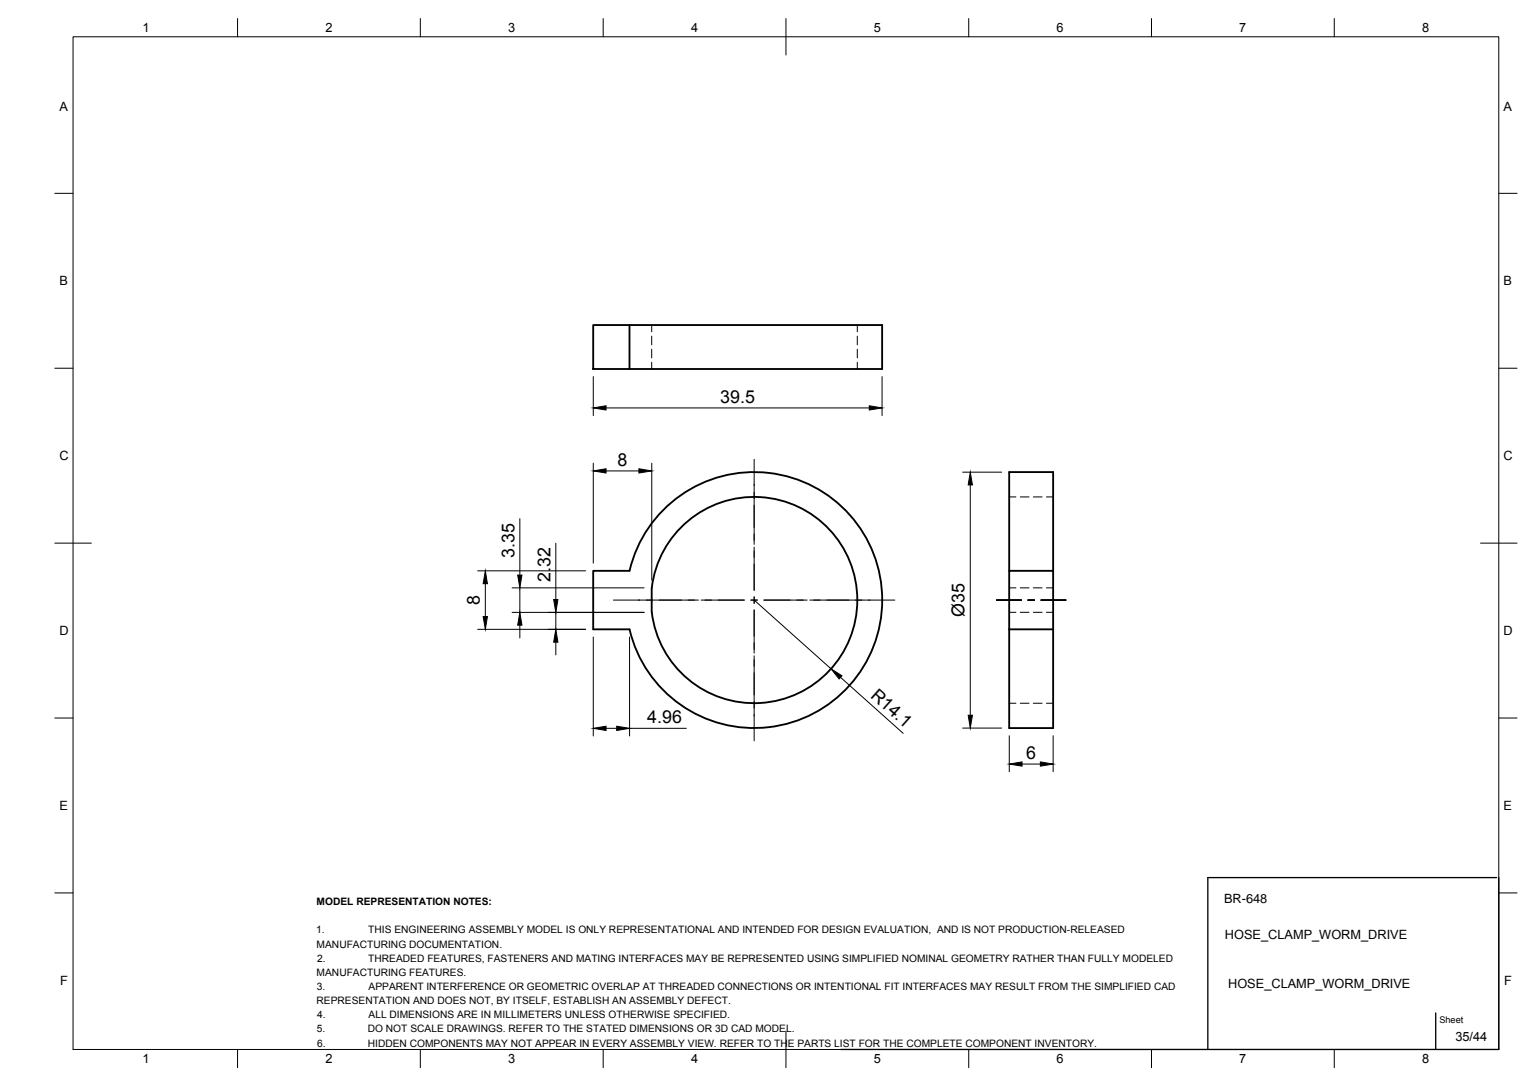
ISO-10303-21;
HEADER;
FILE_DESCRIPTION((''),'2;1');
FILE_NAME('HOSE_CLAMP_WORM_DRIVE.step','2026-10-01T22:05:39-07:00',(''),(''),'','','');
FILE_SCHEMA (('AUTOMOTIVE_DESIGN { 1 0 10303 214 3 1 1 }'));
ENDSEC;
DATA;
#10=MECHANICAL_DESIGN_GEOMETRIC_PRESENTATION_REPRESENTATION('',(#633),#24628);
#549=SHAPE_REPRESENTATION_RELATIONSHIP('SRR','None',#24822,#591) ;
#591=ADVANCED_BREP_SHAPE_REPRESENTATION('',(#672),#24612) ;
#633=STYLED_ITEM('',(#25034),#672) ;
#672=MANIFOLD_SOLID_BREP('HOSE_CLAMP_WORM_DRIVE',#13175) ;
#904=FACE_BOUND('',#4596,.T.) ;
#905=FACE_BOUND('',#4600,.T.) ;
#1679=LINE('',#23705,#2515) ;
#1680=LINE('',#23707,#2516) ;
#1681=LINE('',#23709,#2517) ;
#1682=LINE('',#23710,#2518) ;
#1683=LINE('',#23714,#2519) ;
#1684=LINE('',#23716,#2520) ;
#1685=LINE('',#23718,#2521) ;
#1686=LINE('',#23719,#2522) ;
#1687=LINE('',#23723,#2523) ;
#1688=LINE('',#23725,#2524) ;
#1689=LINE('',#23727,#2525) ;
#1690=LINE('',#23728,#2526) ;
#1691=LINE('',#23730,#2527) ;
#1692=LINE('',#23731,#2528) ;
#2515=VECTOR('',#19054,1.) ;
#2516=VECTOR('',#19055,1.) ;
#2517=VECTOR('',#19056,1.) ;
#2518=VECTOR('',#19057,1.) ;
#2519=VECTOR('',#19060,1.) ;
#2520=VECTOR('',#19061,1.) ;
#2521=VECTOR('',#19062,1.) ;
#2522=VECTOR('',#19063,1.) ;
#2523=VECTOR('',#19066,1.) ;
#2524=VECTOR('',#19067,1.) ;
#2525=VECTOR('',#19068,1.) ;
#2526=VECTOR('',#19069,1.) ;
#2527=VECTOR('',#19072,1.) ;
#2528=VECTOR('',#19073,1.) ;
#2913=CYLINDRICAL_SURFACE('',#15151,1.41) ;
#2914=CYLINDRICAL_SURFACE('',#15153,1.75) ;
#3606=FACE_OUTER_BOUND('',#4591,.T.) ;
#3607=FACE_OUTER_BOUND('',#4592,.T.) ;
#3608=FACE_OUTER_BOUND('',#4593,.T.) ;
#3609=FACE_OUTER_BOUND('',#4594,.T.) ;
#3610=FACE_OUTER_BOUND('',#4595,.T.) ;
#3611=FACE_OUTER_BOUND('',#4597,.T.) ;
#3612=FACE_OUTER_BOUND('',#4598,.T.) ;
#3613=FACE_OUTER_BOUND('',#4599,.T.) ;
#4591=EDGE_LOOP('',(#11495,#11496,#11497,#11498)) ;
#4592=EDGE_LOOP('',(#11499,#11500,#11501,#11502)) ;
#4593=EDGE_LOOP('',(#11503,#11504,#11505,#11506)) ;
#4594=EDGE_LOOP('',(#11507,#11508,#11509,#11510)) ;
#4595=EDGE_LOOP('',(#11511,#11512,#11513,#11514)) ;
#4596=EDGE_LOOP('',(#11515,#11516)) ;
#4597=EDGE_LOOP('',(#11517,#11518,#11519,#11520)) ;
#4598=EDGE_LOOP('',(#11521,#11522,#11523,#11524)) ;
#4599=EDGE_LOOP('',(#11525,#11526,#11527,#11528)) ;
#4600=EDGE_LOOP('',(#11529,#11530)) ;
#5461=CIRCLE('',#15149,1.75) ;
#5462=CIRCLE('',#15150,1.41) ;
#5463=CIRCLE('',#15152,1.41) ;
#5464=CIRCLE('',#15154,1.75) ;
#6567=VERTEX_POINT('',#23703) ;
#6568=VERTEX_POINT('',#23704) ;
#6569=VERTEX_POINT('',#23706) ;
#6570=VERTEX_POINT('',#23708) ;
#6571=VERTEX_POINT('',#23712) ;
#6572=VERTEX_POINT('',#23713) ;
#6573=VERTEX_POINT('',#23715) ;
#6574=VERTEX_POINT('',#23717) ;
#6575=VERTEX_POINT('',#23721) ;
#6576=VERTEX_POINT('',#23722) ;
#6577=VERTEX_POINT('',#23724) ;
#6578=VERTEX_POINT('',#23726) ;
#8237=EDGE_CURVE('',#6567,#6568,#1679,.T.) ;
#8238=EDGE_CURVE('',#6569,#6567,#1680,.T.) ;
#8239=EDGE_CURVE('',#6570,#6569,#1681,.T.) ;
#8240=EDGE_CURVE('',#6568,#6570,#1682,.T.) ;
#8241=EDGE_CURVE('',#6571,#6572,#1683,.T.) ;
#8242=EDGE_CURVE('',#6573,#6571,#1684,.T.) ;
#8243=EDGE_CURVE('',#6574,#6573,#1685,.T.) ;
#8244=EDGE_CURVE('',#6572,#6574,#1686,.T.) ;
#8245=EDGE_CURVE('',#6575,#6576,#1687,.T.) ;
#8246=EDGE_CURVE('',#6577,#6575,#1688,.T.) ;
#8247=EDGE_CURVE('',#6577,#6578,#1689,.T.) ;
#8248=EDGE_CURVE('',#6576,#6578,#1690,.T.) ;
#8249=EDGE_CURVE('',#6578,#6569,#1691,.T.) ;
#8250=EDGE_CURVE('',#6570,#6577,#1692,.T.) ;
#8251=EDGE_CURVE('',#6567,#6576,#5461,.T.) ;
#8252=EDGE_CURVE('',#6574,#6572,#5462,.T.) ;
#8253=EDGE_CURVE('',#6571,#6573,#5463,.T.) ;
#8254=EDGE_CURVE('',#6575,#6568,#5464,.T.) ;
#11495=ORIENTED_EDGE('',*,*,#8237,.F.) ;
#11496=ORIENTED_EDGE('',*,*,#8238,.F.) ;
#11497=ORIENTED_EDGE('',*,*,#8239,.F.) ;
#11498=ORIENTED_EDGE('',*,*,#8240,.F.) ;
#11499=ORIENTED_EDGE('',*,*,#8241,.F.) ;
#11500=ORIENTED_EDGE('',*,*,#8242,.F.) ;
#11501=ORIENTED_EDGE('',*,*,#8243,.F.) ;
#11502=ORIENTED_EDGE('',*,*,#8244,.F.) ;
#11503=ORIENTED_EDGE('',*,*,#8245,.F.) ;
#11504=ORIENTED_EDGE('',*,*,#8246,.F.) ;
#11505=ORIENTED_EDGE('',*,*,#8247,.T.) ;
#11506=ORIENTED_EDGE('',*,*,#8248,.F.) ;
#11507=ORIENTED_EDGE('',*,*,#8239,.T.) ;
#11508=ORIENTED_EDGE('',*,*,#8249,.F.) ;
#11509=ORIENTED_EDGE('',*,*,#8247,.F.) ;
#11510=ORIENTED_EDGE('',*,*,#8250,.F.) ;
#11511=ORIENTED_EDGE('',*,*,#8251,.T.) ;
#11512=ORIENTED_EDGE('',*,*,#8248,.T.) ;
#11513=ORIENTED_EDGE('',*,*,#8249,.T.) ;
#11514=ORIENTED_EDGE('',*,*,#8238,.T.) ;
#11515=ORIENTED_EDGE('',*,*,#8252,.T.) ;
#11516=ORIENTED_EDGE('',*,*,#8244,.T.) ;
#11517=ORIENTED_EDGE('',*,*,#8241,.T.) ;
#11518=ORIENTED_EDGE('',*,*,#8252,.F.) ;
#11519=ORIENTED_EDGE('',*,*,#8243,.T.) ;
#11520=ORIENTED_EDGE('',*,*,#8253,.F.) ;
#11521=ORIENTED_EDGE('',*,*,#8237,.T.) ;
#11522=ORIENTED_EDGE('',*,*,#8254,.F.) ;
#11523=ORIENTED_EDGE('',*,*,#8245,.T.) ;
#11524=ORIENTED_EDGE('',*,*,#8251,.F.) ;
#11525=ORIENTED_EDGE('',*,*,#8240,.T.) ;
#11526=ORIENTED_EDGE('',*,*,#8250,.T.) ;
#11527=ORIENTED_EDGE('',*,*,#8246,.T.) ;
#11528=ORIENTED_EDGE('',*,*,#8254,.T.) ;
#11529=ORIENTED_EDGE('',*,*,#8253,.T.) ;
#11530=ORIENTED_EDGE('',*,*,#8242,.T.) ;
#12275=PLANE('',#15144) ;
#12276=PLANE('',#15145) ;
#12277=PLANE('',#15146) ;
#12278=PLANE('',#15147) ;
#12279=PLANE('',#15148) ;
#12280=PLANE('',#15155) ;
#13001=ADVANCED_FACE('',(#3606),#12275,.F.) ;
#13002=ADVANCED_FACE('',(#3607),#12276,.F.) ;
#13003=ADVANCED_FACE('',(#3608),#12277,.F.) ;
#13004=ADVANCED_FACE('',(#3609),#12278,.F.) ;
#13005=ADVANCED_FACE('',(#3610,#904),#12279,.T.) ;
#13006=ADVANCED_FACE('',(#3611),#2913,.F.) ;
#13007=ADVANCED_FACE('',(#3612),#2914,.T.) ;
#13008=ADVANCED_FACE('',(#3613,#905),#12280,.T.) ;
#13175=CLOSED_SHELL('',(#13001,#13002,#13003,#13004,#13005,#13006,#13007,
#13008)) ;
#15143=AXIS2_PLACEMENT_3D('',#23701,#19050,#19051) ;
#15144=AXIS2_PLACEMENT_3D('',#23702,#19052,#19053) ;
#15145=AXIS2_PLACEMENT_3D('',#23711,#19058,#19059) ;
#15146=AXIS2_PLACEMENT_3D('',#23720,#19064,#19065) ;
#15147=AXIS2_PLACEMENT_3D('',#23729,#19070,#19071) ;
#15148=AXIS2_PLACEMENT_3D('',#23732,#19074,#19075) ;
#15149=AXIS2_PLACEMENT_3D('',#23733,#19076,#19077) ;
#15150=AXIS2_PLACEMENT_3D('',#23734,#19078,#19079) ;
#15151=AXIS2_PLACEMENT_3D('',#23735,#19080,#19081) ;
#15152=AXIS2_PLACEMENT_3D('',#23736,#19082,#19083) ;
#15153=AXIS2_PLACEMENT_3D('',#23737,#19084,#19085) ;
#15154=AXIS2_PLACEMENT_3D('',#23738,#19086,#19087) ;
#15155=AXIS2_PLACEMENT_3D('',#23739,#19088,#19089) ;
#19050=DIRECTION('axis',(0.,0.,1.)) ;
#19051=DIRECTION('refdir',(1.,0.,0.)) ;
#19052=DIRECTION('center_axis',(0.,1.,0.)) ;
#19053=DIRECTION('ref_axis',(0.,0.,1.)) ;
#19054=DIRECTION('',(0.,0.,1.)) ;
#19055=DIRECTION('',(-1.,0.,0.)) ;
#19056=DIRECTION('',(0.,0.,-1.)) ;
#19057=DIRECTION('',(1.,0.,0.)) ;
#19058=DIRECTION('center_axis',(1.,0.,0.)) ;
#19059=DIRECTION('ref_axis',(0.,0.,-1.)) ;
#19060=DIRECTION('',(0.,0.,-1.)) ;
#19061=DIRECTION('',(0.,-1.,0.)) ;
#19062=DIRECTION('',(0.,0.,1.)) ;
#19063=DIRECTION('',(0.,1.,0.)) ;
#19064=DIRECTION('center_axis',(0.,-1.,0.)) ;
#19065=DIRECTION('ref_axis',(0.,0.,-1.)) ;
#19066=DIRECTION('',(0.,0.,-1.)) ;
#19067=DIRECTION('',(-1.,0.,0.)) ;
#19068=DIRECTION('',(0.,0.,-1.)) ;
#19069=DIRECTION('',(1.,0.,0.)) ;
#19070=DIRECTION('center_axis',(-1.,0.,0.)) ;
#19071=DIRECTION('ref_axis',(0.,0.,1.)) ;
#19072=DIRECTION('',(0.,-1.,0.)) ;
#19073=DIRECTION('',(0.,1.,0.)) ;
#19074=DIRECTION('center_axis',(0.,0.,-1.)) ;
#19075=DIRECTION('ref_axis',(-1.,0.,0.)) ;
#19076=DIRECTION('center_axis',(0.,0.,-1.)) ;
#19077=DIRECTION('ref_axis',(1.,0.,0.)) ;
#19078=DIRECTION('center_axis',(0.,0.,1.)) ;
#19079=DIRECTION('ref_axis',(1.,0.,0.)) ;
#19080=DIRECTION('center_axis',(0.,0.,1.)) ;
#19081=DIRECTION('ref_axis',(-1.,-1.22464679914735E-16,0.)) ;
#19082=DIRECTION('center_axis',(0.,0.,-1.)) ;
#19083=DIRECTION('ref_axis',(1.,0.,0.)) ;
#19084=DIRECTION('center_axis',(0.,0.,1.)) ;
#19085=DIRECTION('ref_axis',(-1.,-1.22464679914735E-16,0.)) ;
#19086=DIRECTION('center_axis',(0.,0.,1.)) ;
#19087=DIRECTION('ref_axis',(1.,0.,0.)) ;
#19088=DIRECTION('center_axis',(0.,0.,1.)) ;
#19089=DIRECTION('ref_axis',(1.,0.,0.)) ;
#23701=CARTESIAN_POINT('',(0.,0.,0.)) ;
#23702=CARTESIAN_POINT('Origin',(-21.2,-2.2,-6.9)) ;
#23703=CARTESIAN_POINT('',(-21.2963274962599,-2.2,-7.2)) ;
#23704=CARTESIAN_POINT('',(-21.2963274962599,-2.2,-6.6)) ;
#23705=CARTESIAN_POINT('',(-21.2963274962599,-2.2,-6.9)) ;
#23706=CARTESIAN_POINT('',(-20.8,-2.2,-7.2)) ;
#23707=CARTESIAN_POINT('',(-21.2,-2.2,-7.2)) ;
#23708=CARTESIAN_POINT('',(-20.8,-2.2,-6.6)) ;
#23709=CARTESIAN_POINT('',(-20.8,-2.2,-6.9)) ;
#23710=CARTESIAN_POINT('',(-21.2,-2.2,-6.6)) ;
#23711=CARTESIAN_POINT('Origin',(-21.6,-1.8,-6.9)) ;
#23712=CARTESIAN_POINT('',(-21.6,-1.96763054614242,-6.6)) ;
#23713=CARTESIAN_POINT('',(-21.6,-1.96763054614242,-7.2)) ;
#23714=CARTESIAN_POINT('',(-21.6,-1.96763054614242,-6.9)) ;
#23715=CARTESIAN_POINT('',(-21.6,-1.63236945385758,-6.6)) ;
#23716=CARTESIAN_POINT('',(-21.6,-1.8,-6.6)) ;
#23717=CARTESIAN_POINT('',(-21.6,-1.63236945385758,-7.2)) ;
#23718=CARTESIAN_POINT('',(-21.6,-1.63236945385758,-6.9)) ;
#23719=CARTESIAN_POINT('',(-21.6,-1.8,-7.2)) ;
#23720=CARTESIAN_POINT('Origin',(-21.2,-1.4,-6.9)) ;
#23721=CARTESIAN_POINT('',(-21.2963274962599,-1.4,-6.6)) ;
#23722=CARTESIAN_POINT('',(-21.2963274962599,-1.4,-7.2)) ;
#23723=CARTESIAN_POINT('',(-21.2963274962599,-1.4,-6.9)) ;
#23724=CARTESIAN_POINT('',(-20.8,-1.4,-6.6)) ;
#23725=CARTESIAN_POINT('',(-21.2,-1.4,-6.6)) ;
#23726=CARTESIAN_POINT('',(-20.8,-1.4,-7.2)) ;
#23727=CARTESIAN_POINT('',(-20.8,-1.4,-6.9)) ;
#23728=CARTESIAN_POINT('',(-21.2,-1.4,-7.2)) ;
#23729=CARTESIAN_POINT('Origin',(-20.8,-1.8,-6.9)) ;
#23730=CARTESIAN_POINT('',(-20.8,-1.8,-7.2)) ;
#23731=CARTESIAN_POINT('',(-20.8,-1.8,-6.6)) ;
#23732=CARTESIAN_POINT('Origin',(-23.,-1.8,-7.2)) ;
#23733=CARTESIAN_POINT('Origin',(-23.,-1.8,-7.2)) ;
#23734=CARTESIAN_POINT('Origin',(-23.,-1.8,-7.2)) ;
#23735=CARTESIAN_POINT('Origin',(-23.,-1.8,-6.9)) ;
#23736=CARTESIAN_POINT('Origin',(-23.,-1.8,-6.6)) ;
#23737=CARTESIAN_POINT('Origin',(-23.,-1.8,-6.9)) ;
#23738=CARTESIAN_POINT('Origin',(-23.,-1.8,-6.6)) ;
#23739=CARTESIAN_POINT('Origin',(-23.,-1.8,-6.6)) ;
#24564=UNCERTAINTY_MEASURE_WITH_UNIT(LENGTH_MEASURE(0.001),#24629,
'DISTANCE_ACCURACY_VALUE',
'Maximum model space distance between geometric entities at asserted c
onnectivities') ;
#24580=UNCERTAINTY_MEASURE_WITH_UNIT(LENGTH_MEASURE(0.001),#24629,
'DISTANCE_ACCURACY_VALUE',
'Maximum model space distance between geometric entities at asserted c
onnectivities') ;
#24612=(
GEOMETRIC_REPRESENTATION_CONTEXT(3)
GLOBAL_UNCERTAINTY_ASSIGNED_CONTEXT((#24564))
GLOBAL_UNIT_ASSIGNED_CONTEXT((#24629,#24631,#24632))
REPRESENTATION_CONTEXT('','3D')
) ;
#24628=(
GEOMETRIC_REPRESENTATION_CONTEXT(3)
GLOBAL_UNCERTAINTY_ASSIGNED_CONTEXT((#24580))
GLOBAL_UNIT_ASSIGNED_CONTEXT((#24629,#24631,#24632))
REPRESENTATION_CONTEXT('','3D')
) ;
#24629=(
LENGTH_UNIT()
NAMED_UNIT(*)
SI_UNIT(.CENTI.,.METRE.)
) ;
#24631=(
NAMED_UNIT(*)
PLANE_ANGLE_UNIT()
SI_UNIT($,.RADIAN.)
) ;
#24632=(
NAMED_UNIT(*)
SI_UNIT($,.STERADIAN.)
SOLID_ANGLE_UNIT()
) ;
#24664=SHAPE_DEFINITION_REPRESENTATION(#24733,#24822) ;
#24733=PRODUCT_DEFINITION_SHAPE('',$,#24870) ;
#24822=SHAPE_REPRESENTATION('',(#15143),#24612) ;
#24838=PRODUCT_DEFINITION_CONTEXT('part definition',#24981,'design') ;
#24870=PRODUCT_DEFINITION('HOSE_CLAMP_WORM_DRIVE',
'HOSE_CLAMP_WORM_DRIVE',#24917,#24838) ;
#24917=PRODUCT_DEFINITION_FORMATION('',$,#25014) ;
#24981=APPLICATION_CONTEXT(
'Core Data for Automotive Mechanical Design Process') ;
#24982=PRODUCT_CONTEXT('part definition',#24981,'mechanical') ;
#25014=PRODUCT('HOSE_CLAMP_WORM_DRIVE','HOSE_CLAMP_WORM_DRIVE',$,(#24982)) ;
#25034=PRESENTATION_STYLE_ASSIGNMENT((#25044)) ;
#25044=SURFACE_STYLE_USAGE(.BOTH.,#25054) ;
#25054=SURFACE_SIDE_STYLE('',(#25064)) ;
#25064=SURFACE_STYLE_FILL_AREA(#25074) ;
#25074=FILL_AREA_STYLE('Stainless Steel - Satin',(#25084)) ;
#25084=FILL_AREA_STYLE_COLOUR('Stainless Steel - Satin',#25094) ;
#25094=COLOUR_RGB('Stainless Steel - Satin', 0.31764706, 0.68627451, 0.89019608) ;
ENDSEC;
END-ISO-10303-21;
